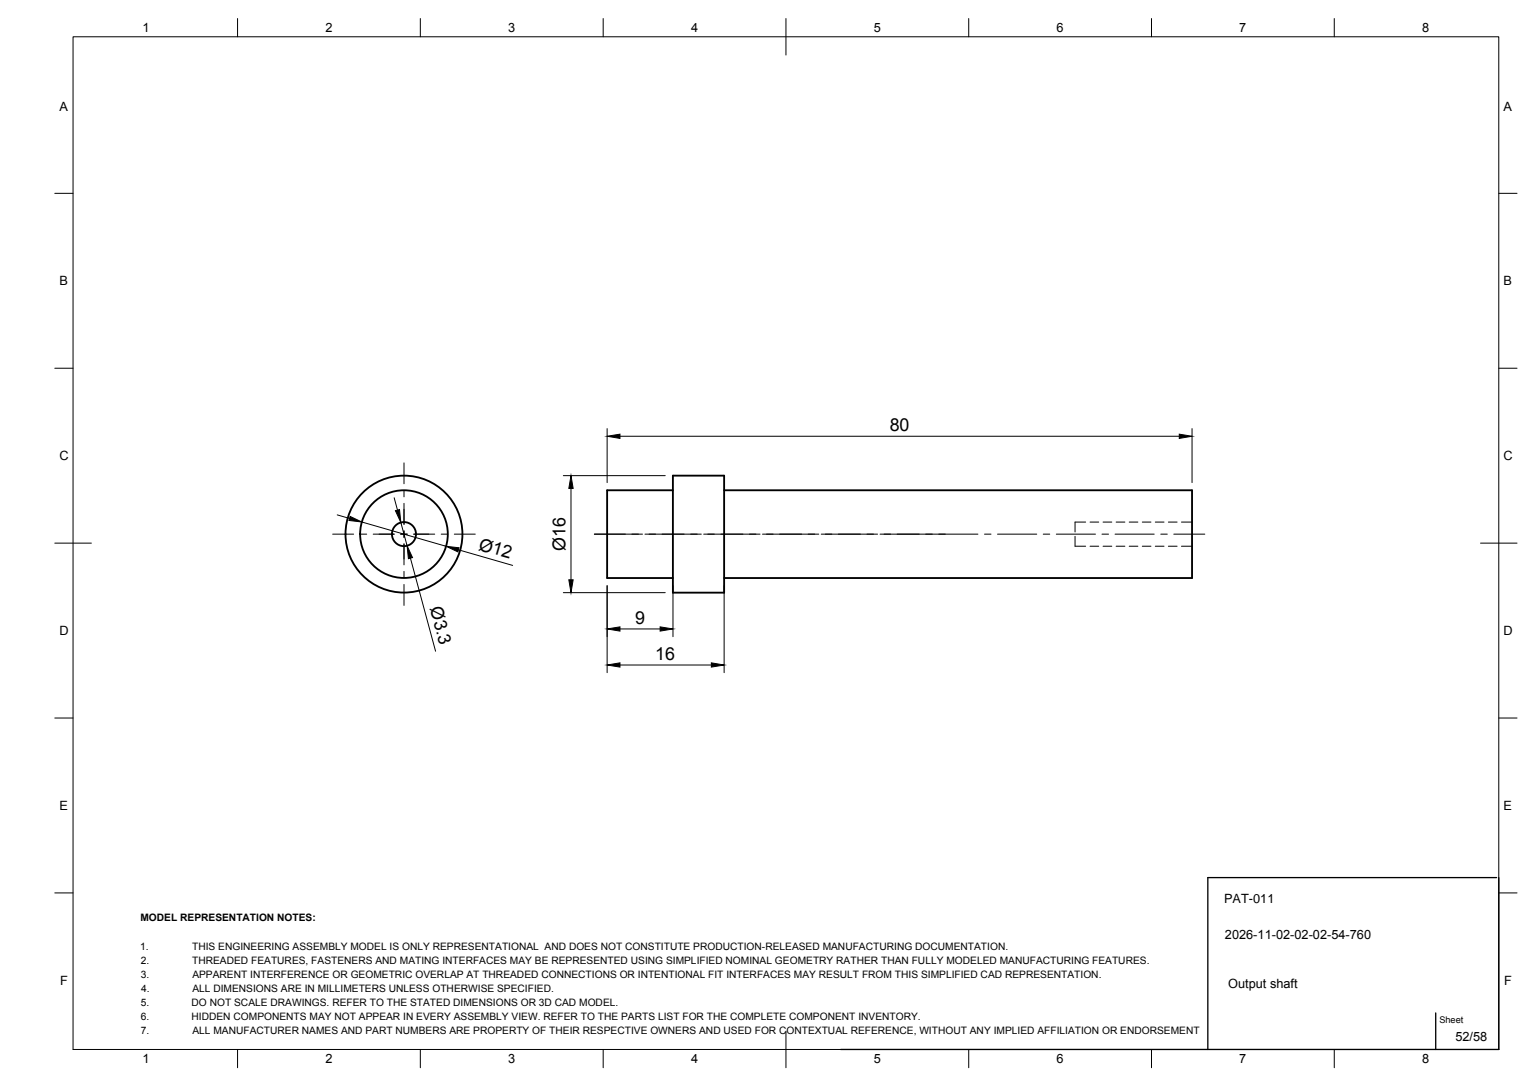
ISO-10303-21;
HEADER;
/* Generated by software containing ST-Developer
 * from STEP Tools, Inc. (www.steptools.com) 
 */

FILE_DESCRIPTION(
/* description */ ('Belt tension measurement rig'),
/* implementation_level */ '2;1');

FILE_NAME(
/* name */ 'Output shaft.step',
/* time_stamp */ '2026-10-28T03:24:44-07:00',
/* author */ (''),
/* organization */ (''),
/* preprocessor_version */ 'ST-DEVELOPER v20.2',
/* originating_system */ 'Autodesk Translation Framework v15.17.0.0',
/* authorisation */ '');

FILE_SCHEMA (('AUTOMOTIVE_DESIGN { 1 0 10303 214 3 1 1 }'));
ENDSEC;

DATA;
#10=MECHANICAL_DESIGN_GEOMETRIC_PRESENTATION_REPRESENTATION('',(#751),#23587);
#626=SHAPE_REPRESENTATION_RELATIONSHIP('SRR','None',#23877,#681);
#681=ADVANCED_BREP_SHAPE_REPRESENTATION('',(#819),#23575);
#751=STYLED_ITEM('',(#24211),#819);
#819=MANIFOLD_SOLID_BREP('Body1',#12258);
#1006=FACE_BOUND('',#2767,.T.);
#1007=FACE_BOUND('',#2769,.T.);
#1008=FACE_BOUND('',#2773,.T.);
#1299=PLANE('',#14018);
#1300=PLANE('',#14019);
#1301=PLANE('',#14022);
#1302=PLANE('',#14028);
#1303=PLANE('',#14031);
#1883=FACE_OUTER_BOUND('',#2764,.T.);
#1884=FACE_OUTER_BOUND('',#2765,.T.);
#1885=FACE_OUTER_BOUND('',#2766,.T.);
#1886=FACE_OUTER_BOUND('',#2768,.T.);
#1887=FACE_OUTER_BOUND('',#2770,.T.);
#1888=FACE_OUTER_BOUND('',#2771,.T.);
#1889=FACE_OUTER_BOUND('',#2772,.T.);
#1890=FACE_OUTER_BOUND('',#2774,.T.);
#1891=FACE_OUTER_BOUND('',#2775,.T.);
#2764=EDGE_LOOP('',(#10324,#10325,#10326,#10327));
#2765=EDGE_LOOP('',(#10328));
#2766=EDGE_LOOP('',(#10329));
#2767=EDGE_LOOP('',(#10330));
#2768=EDGE_LOOP('',(#10331));
#2769=EDGE_LOOP('',(#10332));
#2770=EDGE_LOOP('',(#10333,#10334,#10335,#10336));
#2771=EDGE_LOOP('',(#10337,#10338,#10339,#10340));
#2772=EDGE_LOOP('',(#10341));
#2773=EDGE_LOOP('',(#10342));
#2774=EDGE_LOOP('',(#10343,#10344,#10345,#10346));
#2775=EDGE_LOOP('',(#10347));
#3557=LINE('',#22157,#4308);
#3558=LINE('',#22171,#4309);
#3559=LINE('',#22174,#4310);
#3560=LINE('',#22180,#4311);
#4308=VECTOR('',#17388,0.164999999999999);
#4309=VECTOR('',#17407,0.800000000000001);
#4310=VECTOR('',#17410,0.6);
#4311=VECTOR('',#17419,0.6);
#5012=CIRCLE('',#14016,0.164999999999999);
#5013=CIRCLE('',#14017,0.164999999999999);
#5014=CIRCLE('',#14020,0.800000000000001);
#5015=CIRCLE('',#14021,0.6);
#5016=CIRCLE('',#14023,0.800000000000001);
#5017=CIRCLE('',#14024,0.6);
#5018=CIRCLE('',#14027,0.6);
#5019=CIRCLE('',#14030,0.6);
#6049=VERTEX_POINT('',#22154);
#6050=VERTEX_POINT('',#22156);
#6051=VERTEX_POINT('',#22161);
#6052=VERTEX_POINT('',#22163);
#6053=VERTEX_POINT('',#22166);
#6054=VERTEX_POINT('',#22168);
#6055=VERTEX_POINT('',#22173);
#6056=VERTEX_POINT('',#22178);
#7521=EDGE_CURVE('',#6049,#6049,#5012,.T.);
#7522=EDGE_CURVE('',#6049,#6050,#3557,.T.);
#7523=EDGE_CURVE('',#6050,#6050,#5013,.T.);
#7524=EDGE_CURVE('',#6051,#6051,#5014,.T.);
#7525=EDGE_CURVE('',#6052,#6052,#5015,.T.);
#7526=EDGE_CURVE('',#6053,#6053,#5016,.T.);
#7527=EDGE_CURVE('',#6054,#6054,#5017,.T.);
#7528=EDGE_CURVE('',#6051,#6053,#3558,.T.);
#7529=EDGE_CURVE('',#6054,#6055,#3559,.T.);
#7530=EDGE_CURVE('',#6055,#6055,#5018,.T.);
#7531=EDGE_CURVE('',#6056,#6056,#5019,.T.);
#7532=EDGE_CURVE('',#6056,#6052,#3560,.T.);
#10324=ORIENTED_EDGE('',*,*,#7521,.F.);
#10325=ORIENTED_EDGE('',*,*,#7522,.T.);
#10326=ORIENTED_EDGE('',*,*,#7523,.T.);
#10327=ORIENTED_EDGE('',*,*,#7522,.F.);
#10328=ORIENTED_EDGE('',*,*,#7523,.F.);
#10329=ORIENTED_EDGE('',*,*,#7524,.T.);
#10330=ORIENTED_EDGE('',*,*,#7525,.F.);
#10331=ORIENTED_EDGE('',*,*,#7526,.F.);
#10332=ORIENTED_EDGE('',*,*,#7527,.F.);
#10333=ORIENTED_EDGE('',*,*,#7524,.F.);
#10334=ORIENTED_EDGE('',*,*,#7528,.T.);
#10335=ORIENTED_EDGE('',*,*,#7526,.T.);
#10336=ORIENTED_EDGE('',*,*,#7528,.F.);
#10337=ORIENTED_EDGE('',*,*,#7527,.T.);
#10338=ORIENTED_EDGE('',*,*,#7529,.T.);
#10339=ORIENTED_EDGE('',*,*,#7530,.T.);
#10340=ORIENTED_EDGE('',*,*,#7529,.F.);
#10341=ORIENTED_EDGE('',*,*,#7530,.F.);
#10342=ORIENTED_EDGE('',*,*,#7521,.T.);
#10343=ORIENTED_EDGE('',*,*,#7531,.F.);
#10344=ORIENTED_EDGE('',*,*,#7532,.T.);
#10345=ORIENTED_EDGE('',*,*,#7525,.T.);
#10346=ORIENTED_EDGE('',*,*,#7532,.F.);
#10347=ORIENTED_EDGE('',*,*,#7531,.T.);
#11379=CYLINDRICAL_SURFACE('',#14015,0.164999999999999);
#11380=CYLINDRICAL_SURFACE('',#14025,0.800000000000001);
#11381=CYLINDRICAL_SURFACE('',#14026,0.6);
#11382=CYLINDRICAL_SURFACE('',#14029,0.6);
#12024=ADVANCED_FACE('',(#1883),#11379,.F.);
#12025=ADVANCED_FACE('',(#1884),#1299,.F.);
#12026=ADVANCED_FACE('',(#1885,#1006),#1300,.T.);
#12027=ADVANCED_FACE('',(#1886,#1007),#1301,.F.);
#12028=ADVANCED_FACE('',(#1887),#11380,.T.);
#12029=ADVANCED_FACE('',(#1888),#11381,.T.);
#12030=ADVANCED_FACE('',(#1889,#1008),#1302,.F.);
#12031=ADVANCED_FACE('',(#1890),#11382,.T.);
#12032=ADVANCED_FACE('',(#1891),#1303,.T.);
#12258=CLOSED_SHELL('',(#12024,#12025,#12026,#12027,#12028,#12029,#12030,
#12031,#12032));
#14014=AXIS2_PLACEMENT_3D('',#22152,#17382,#17383);
#14015=AXIS2_PLACEMENT_3D('',#22153,#17384,#17385);
#14016=AXIS2_PLACEMENT_3D('',#22155,#17386,#17387);
#14017=AXIS2_PLACEMENT_3D('',#22158,#17389,#17390);
#14018=AXIS2_PLACEMENT_3D('',#22159,#17391,#17392);
#14019=AXIS2_PLACEMENT_3D('',#22160,#17393,#17394);
#14020=AXIS2_PLACEMENT_3D('',#22162,#17395,#17396);
#14021=AXIS2_PLACEMENT_3D('',#22164,#17397,#17398);
#14022=AXIS2_PLACEMENT_3D('',#22165,#17399,#17400);
#14023=AXIS2_PLACEMENT_3D('',#22167,#17401,#17402);
#14024=AXIS2_PLACEMENT_3D('',#22169,#17403,#17404);
#14025=AXIS2_PLACEMENT_3D('',#22170,#17405,#17406);
#14026=AXIS2_PLACEMENT_3D('',#22172,#17408,#17409);
#14027=AXIS2_PLACEMENT_3D('',#22175,#17411,#17412);
#14028=AXIS2_PLACEMENT_3D('',#22176,#17413,#17414);
#14029=AXIS2_PLACEMENT_3D('',#22177,#17415,#17416);
#14030=AXIS2_PLACEMENT_3D('',#22179,#17417,#17418);
#14031=AXIS2_PLACEMENT_3D('',#22181,#17420,#17421);
#17382=DIRECTION('axis',(0.,0.,1.));
#17383=DIRECTION('refdir',(1.,0.,0.));
#17384=DIRECTION('center_axis',(0.,1.,0.));
#17385=DIRECTION('ref_axis',(1.,0.,0.));
#17386=DIRECTION('center_axis',(0.,1.,0.));
#17387=DIRECTION('ref_axis',(1.,0.,0.));
#17388=DIRECTION('',(0.,1.,0.));
#17389=DIRECTION('center_axis',(0.,1.,0.));
#17390=DIRECTION('ref_axis',(1.,0.,0.));
#17391=DIRECTION('center_axis',(0.,1.,0.));
#17392=DIRECTION('ref_axis',(1.,0.,0.));
#17393=DIRECTION('center_axis',(0.,1.,0.));
#17394=DIRECTION('ref_axis',(1.,0.,0.));
#17395=DIRECTION('center_axis',(0.,1.,0.));
#17396=DIRECTION('ref_axis',(1.,0.,0.));
#17397=DIRECTION('center_axis',(0.,1.,0.));
#17398=DIRECTION('ref_axis',(1.,0.,0.));
#17399=DIRECTION('center_axis',(0.,1.,0.));
#17400=DIRECTION('ref_axis',(1.,0.,0.));
#17401=DIRECTION('center_axis',(0.,1.,0.));
#17402=DIRECTION('ref_axis',(1.,0.,0.));
#17403=DIRECTION('center_axis',(0.,-1.,0.));
#17404=DIRECTION('ref_axis',(1.,0.,0.));
#17405=DIRECTION('center_axis',(0.,1.,0.));
#17406=DIRECTION('ref_axis',(1.,0.,0.));
#17407=DIRECTION('',(0.,-1.,0.));
#17408=DIRECTION('center_axis',(0.,1.,0.));
#17409=DIRECTION('ref_axis',(1.,0.,0.));
#17410=DIRECTION('',(0.,-1.,0.));
#17411=DIRECTION('center_axis',(0.,1.,0.));
#17412=DIRECTION('ref_axis',(1.,0.,0.));
#17413=DIRECTION('center_axis',(0.,1.,0.));
#17414=DIRECTION('ref_axis',(1.,0.,0.));
#17415=DIRECTION('center_axis',(0.,1.,0.));
#17416=DIRECTION('ref_axis',(1.,0.,0.));
#17417=DIRECTION('center_axis',(0.,1.,0.));
#17418=DIRECTION('ref_axis',(1.,0.,0.));
#17419=DIRECTION('',(0.,-1.,0.));
#17420=DIRECTION('center_axis',(0.,1.,0.));
#17421=DIRECTION('ref_axis',(1.,0.,0.));
#22152=CARTESIAN_POINT('',(0.,0.,0.));
#22153=CARTESIAN_POINT('Origin',(10.,-5.1,7.));
#22154=CARTESIAN_POINT('',(9.835,-5.,7.));
#22155=CARTESIAN_POINT('Origin',(10.,-5.,7.));
#22156=CARTESIAN_POINT('',(9.835,-3.4,7.));
#22157=CARTESIAN_POINT('',(9.835,-5.1,7.));
#22158=CARTESIAN_POINT('Origin',(10.,-3.4,7.));
#22159=CARTESIAN_POINT('Origin',(10.,-3.4,7.));
#22160=CARTESIAN_POINT('Origin',(10.,2.1,7.));
#22161=CARTESIAN_POINT('',(9.2,2.1,7.));
#22162=CARTESIAN_POINT('Origin',(10.,2.1,7.));
#22163=CARTESIAN_POINT('',(9.4,2.1,7.));
#22164=CARTESIAN_POINT('Origin',(10.,2.1,7.));
#22165=CARTESIAN_POINT('Origin',(10.,1.4,7.));
#22166=CARTESIAN_POINT('',(9.2,1.4,7.));
#22167=CARTESIAN_POINT('Origin',(10.,1.4,7.));
#22168=CARTESIAN_POINT('',(9.4,1.4,7.));
#22169=CARTESIAN_POINT('Origin',(10.,1.4,7.));
#22170=CARTESIAN_POINT('Origin',(10.,1.4,7.));
#22171=CARTESIAN_POINT('',(9.2,1.4,7.));
#22172=CARTESIAN_POINT('Origin',(10.,-1.8,7.));
#22173=CARTESIAN_POINT('',(9.4,-5.,7.));
#22174=CARTESIAN_POINT('',(9.4,-1.8,7.));
#22175=CARTESIAN_POINT('Origin',(10.,-5.,7.));
#22176=CARTESIAN_POINT('Origin',(10.,-5.,7.));
#22177=CARTESIAN_POINT('Origin',(10.,-1.8,7.));
#22178=CARTESIAN_POINT('',(9.4,3.,7.));
#22179=CARTESIAN_POINT('Origin',(10.,3.,7.));
#22180=CARTESIAN_POINT('',(9.4,-1.8,7.));
#22181=CARTESIAN_POINT('Origin',(10.,3.,7.));
#23510=UNCERTAINTY_MEASURE_WITH_UNIT(LENGTH_MEASURE(0.001),#23588,
'DISTANCE_ACCURACY_VALUE',
'Maximum model space distance between geometric entities at asserted c
onnectivities');
#23522=UNCERTAINTY_MEASURE_WITH_UNIT(LENGTH_MEASURE(0.001),#23588,
'DISTANCE_ACCURACY_VALUE',
'Maximum model space distance between geometric entities at asserted c
onnectivities');
#23575=(
GEOMETRIC_REPRESENTATION_CONTEXT(3)
GLOBAL_UNCERTAINTY_ASSIGNED_CONTEXT((#23510))
GLOBAL_UNIT_ASSIGNED_CONTEXT((#23588,#23590,#23591))
REPRESENTATION_CONTEXT('','3D')
);
#23587=(
GEOMETRIC_REPRESENTATION_CONTEXT(3)
GLOBAL_UNCERTAINTY_ASSIGNED_CONTEXT((#23522))
GLOBAL_UNIT_ASSIGNED_CONTEXT((#23588,#23590,#23591))
REPRESENTATION_CONTEXT('','3D')
);
#23588=(
LENGTH_UNIT()
NAMED_UNIT(*)
SI_UNIT(.CENTI.,.METRE.)
);
#23590=(
NAMED_UNIT(*)
PLANE_ANGLE_UNIT()
SI_UNIT($,.RADIAN.)
);
#23591=(
NAMED_UNIT(*)
SI_UNIT($,.STERADIAN.)
SOLID_ANGLE_UNIT()
);
#23644=SHAPE_DEFINITION_REPRESENTATION(#23721,#23877);
#23721=PRODUCT_DEFINITION_SHAPE('',$,#23942);
#23877=SHAPE_REPRESENTATION('',(#14014),#23575);
#23889=PRODUCT_DEFINITION_CONTEXT('part definition',#24083,'design');
#23942=PRODUCT_DEFINITION('Output shaft','Output shaft',#24006,#23889);
#24006=PRODUCT_DEFINITION_FORMATION('',$,#24137);
#24083=APPLICATION_CONTEXT(
'Core Data for Automotive Mechanical Design Process');
#24084=PRODUCT_CONTEXT('part definition',#24083,'mechanical');
#24137=PRODUCT('Output shaft','Output shaft','Output shaft',(#24084));
#24205=COLOUR_RGB('Grey',0.48,0.52,0.57);
#24206=FILL_AREA_STYLE_COLOUR('',#24205);
#24207=FILL_AREA_STYLE('',(#24206));
#24208=SURFACE_STYLE_FILL_AREA(#24207);
#24209=SURFACE_SIDE_STYLE('',(#24208));
#24210=SURFACE_STYLE_USAGE(.BOTH.,#24209);
#24211=PRESENTATION_STYLE_ASSIGNMENT((#24210));
ENDSEC;
END-ISO-10303-21;
